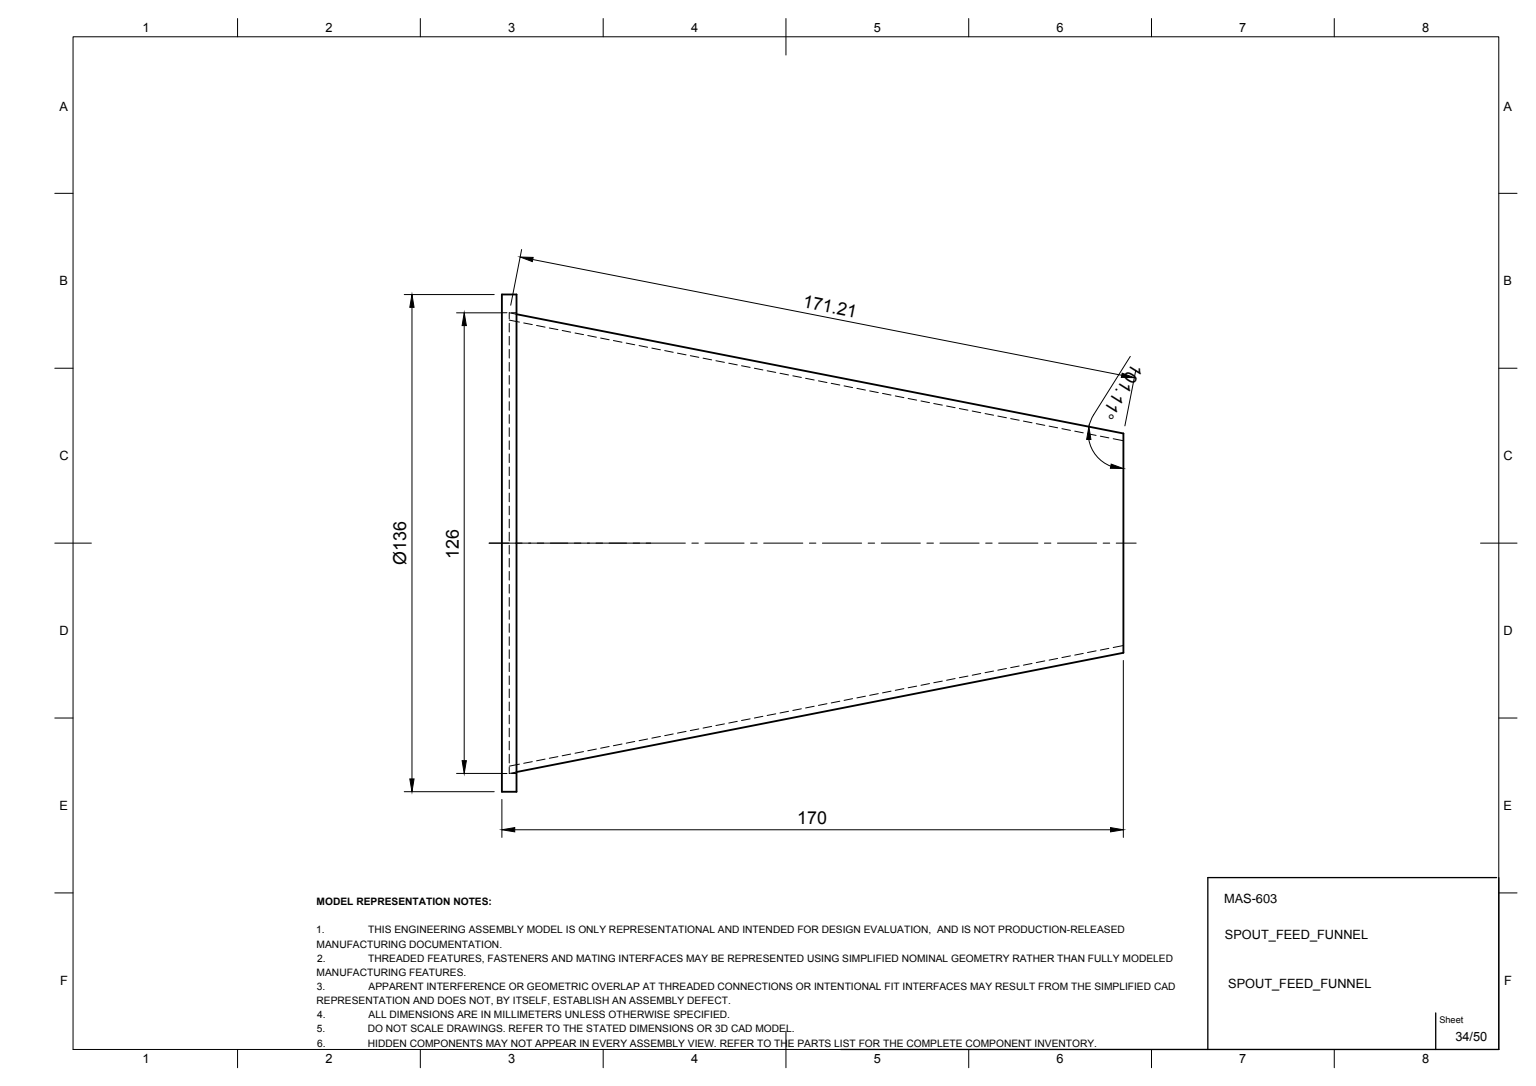
ISO-10303-21;
HEADER;
FILE_DESCRIPTION((''),'2;1');
FILE_NAME('SPOUT_FEED_FUNNEL.step','2026-10-01T22:06:14-07:00',(''),(''),'','','');
FILE_SCHEMA (('AUTOMOTIVE_DESIGN { 1 0 10303 214 3 1 1 }'));
ENDSEC;
DATA;
#10=MECHANICAL_DESIGN_GEOMETRIC_PRESENTATION_REPRESENTATION('',(#1006,#1007),#50440);
#914=SHAPE_REPRESENTATION_RELATIONSHIP('SRR','None',#50647,#959) ;
#959=ADVANCED_BREP_SHAPE_REPRESENTATION('',(#1061,#1062),#50416) ;
#1006=STYLED_ITEM('',(#50889),#1061) ;
#1007=STYLED_ITEM('',(#50889),#1062) ;
#1061=MANIFOLD_SOLID_BREP('SPOUT_FEED_FUNNEL',#28673) ;
#1062=MANIFOLD_SOLID_BREP('SPOUT_FEED_FUNNEL',#28674) ;
#1094=CONICAL_SURFACE('',#30858,4.65,0.193959147259893) ;
#1095=CONICAL_SURFACE('',#30859,4.45,0.193959147259893) ;
#1350=FACE_BOUND('',#5163,.T.) ;
#1351=FACE_BOUND('',#5165,.T.) ;
#1352=FACE_BOUND('',#5167,.T.) ;
#1353=FACE_BOUND('',#5169,.T.) ;
#2201=PLANE('',#30850) ;
#2202=PLANE('',#30851) ;
#2203=PLANE('',#30852) ;
#2204=PLANE('',#30855) ;
#3367=FACE_OUTER_BOUND('',#5159,.T.) ;
#3368=FACE_OUTER_BOUND('',#5160,.T.) ;
#3369=FACE_OUTER_BOUND('',#5161,.T.) ;
#3370=FACE_OUTER_BOUND('',#5162,.T.) ;
#3371=FACE_OUTER_BOUND('',#5164,.T.) ;
#3372=FACE_OUTER_BOUND('',#5166,.T.) ;
#3373=FACE_OUTER_BOUND('',#5168,.T.) ;
#3374=FACE_OUTER_BOUND('',#5170,.T.) ;
#3375=FACE_OUTER_BOUND('',#5171,.T.) ;
#5159=EDGE_LOOP('',(#23895,#23896,#23897,#23898)) ;
#5160=EDGE_LOOP('',(#23899,#23900,#23901,#23902)) ;
#5161=EDGE_LOOP('',(#23903,#23904,#23905,#23906)) ;
#5162=EDGE_LOOP('',(#23907)) ;
#5163=EDGE_LOOP('',(#23908)) ;
#5164=EDGE_LOOP('',(#23909)) ;
#5165=EDGE_LOOP('',(#23910)) ;
#5166=EDGE_LOOP('',(#23911)) ;
#5167=EDGE_LOOP('',(#23912)) ;
#5168=EDGE_LOOP('',(#23913)) ;
#5169=EDGE_LOOP('',(#23914)) ;
#5170=EDGE_LOOP('',(#23915,#23916,#23917,#23918)) ;
#5171=EDGE_LOOP('',(#23919,#23920,#23921,#23922)) ;
#7819=LINE('',#46974,#10291) ;
#7820=LINE('',#46978,#10292) ;
#7821=LINE('',#46984,#10293) ;
#7822=LINE('',#46999,#10294) ;
#7823=LINE('',#47001,#10295) ;
#10291=VECTOR('',#37732,6.3) ;
#10292=VECTOR('',#37737,6.3) ;
#10293=VECTOR('',#37744,6.8) ;
#10294=VECTOR('',#37765,4.65) ;
#10295=VECTOR('',#37768,4.45) ;
#11196=CIRCLE('',#30843,6.3) ;
#11197=CIRCLE('',#30844,6.3) ;
#11198=CIRCLE('',#30846,6.3) ;
#11199=CIRCLE('',#30848,6.8) ;
#11200=CIRCLE('',#30849,6.8) ;
#11201=CIRCLE('',#30853,3.) ;
#11202=CIRCLE('',#30854,2.8) ;
#11203=CIRCLE('',#30856,6.3) ;
#11204=CIRCLE('',#30857,6.1) ;
#13614=VERTEX_POINT('',#46971) ;
#13615=VERTEX_POINT('',#46973) ;
#13616=VERTEX_POINT('',#46977) ;
#13617=VERTEX_POINT('',#46981) ;
#13618=VERTEX_POINT('',#46983) ;
#13619=VERTEX_POINT('',#46989) ;
#13620=VERTEX_POINT('',#46991) ;
#13621=VERTEX_POINT('',#46994) ;
#13622=VERTEX_POINT('',#46996) ;
#17213=EDGE_CURVE('',#13614,#13614,#11196,.T.) ;
#17214=EDGE_CURVE('',#13614,#13615,#7819,.T.) ;
#17215=EDGE_CURVE('',#13615,#13615,#11197,.T.) ;
#17216=EDGE_CURVE('',#13615,#13616,#7820,.T.) ;
#17217=EDGE_CURVE('',#13616,#13616,#11198,.T.) ;
#17218=EDGE_CURVE('',#13617,#13617,#11199,.T.) ;
#17219=EDGE_CURVE('',#13617,#13618,#7821,.T.) ;
#17220=EDGE_CURVE('',#13618,#13618,#11200,.T.) ;
#17221=EDGE_CURVE('',#13619,#13619,#11201,.T.) ;
#17222=EDGE_CURVE('',#13620,#13620,#11202,.T.) ;
#17223=EDGE_CURVE('',#13621,#13621,#11203,.T.) ;
#17224=EDGE_CURVE('',#13622,#13622,#11204,.T.) ;
#17225=EDGE_CURVE('',#13619,#13621,#7822,.T.) ;
#17226=EDGE_CURVE('',#13622,#13620,#7823,.T.) ;
#23895=ORIENTED_EDGE('',*,*,#17213,.F.) ;
#23896=ORIENTED_EDGE('',*,*,#17214,.T.) ;
#23897=ORIENTED_EDGE('',*,*,#17215,.T.) ;
#23898=ORIENTED_EDGE('',*,*,#17214,.F.) ;
#23899=ORIENTED_EDGE('',*,*,#17215,.F.) ;
#23900=ORIENTED_EDGE('',*,*,#17216,.T.) ;
#23901=ORIENTED_EDGE('',*,*,#17217,.F.) ;
#23902=ORIENTED_EDGE('',*,*,#17216,.F.) ;
#23903=ORIENTED_EDGE('',*,*,#17218,.F.) ;
#23904=ORIENTED_EDGE('',*,*,#17219,.T.) ;
#23905=ORIENTED_EDGE('',*,*,#17220,.F.) ;
#23906=ORIENTED_EDGE('',*,*,#17219,.F.) ;
#23907=ORIENTED_EDGE('',*,*,#17220,.T.) ;
#23908=ORIENTED_EDGE('',*,*,#17213,.T.) ;
#23909=ORIENTED_EDGE('',*,*,#17218,.T.) ;
#23910=ORIENTED_EDGE('',*,*,#17217,.T.) ;
#23911=ORIENTED_EDGE('',*,*,#17221,.T.) ;
#23912=ORIENTED_EDGE('',*,*,#17222,.T.) ;
#23913=ORIENTED_EDGE('',*,*,#17223,.T.) ;
#23914=ORIENTED_EDGE('',*,*,#17224,.T.) ;
#23915=ORIENTED_EDGE('',*,*,#17221,.F.) ;
#23916=ORIENTED_EDGE('',*,*,#17225,.T.) ;
#23917=ORIENTED_EDGE('',*,*,#17223,.F.) ;
#23918=ORIENTED_EDGE('',*,*,#17225,.F.) ;
#23919=ORIENTED_EDGE('',*,*,#17224,.F.) ;
#23920=ORIENTED_EDGE('',*,*,#17226,.T.) ;
#23921=ORIENTED_EDGE('',*,*,#17222,.F.) ;
#23922=ORIENTED_EDGE('',*,*,#17226,.F.) ;
#26853=CYLINDRICAL_SURFACE('',#30842,6.3) ;
#26854=CYLINDRICAL_SURFACE('',#30845,6.3) ;
#26855=CYLINDRICAL_SURFACE('',#30847,6.8) ;
#28102=ADVANCED_FACE('',(#3367),#26853,.F.) ;
#28103=ADVANCED_FACE('',(#3368),#26854,.F.) ;
#28104=ADVANCED_FACE('',(#3369),#26855,.T.) ;
#28105=ADVANCED_FACE('',(#3370,#1350),#2201,.T.) ;
#28106=ADVANCED_FACE('',(#3371,#1351),#2202,.T.) ;
#28107=ADVANCED_FACE('',(#3372,#1352),#2203,.T.) ;
#28108=ADVANCED_FACE('',(#3373,#1353),#2204,.T.) ;
#28109=ADVANCED_FACE('',(#3374),#1094,.T.) ;
#28110=ADVANCED_FACE('',(#3375),#1095,.F.) ;
#28673=CLOSED_SHELL('',(#28102,#28103,#28104,#28105,#28106)) ;
#28674=CLOSED_SHELL('',(#28107,#28108,#28109,#28110)) ;
#30841=AXIS2_PLACEMENT_3D('',#46969,#37726,#37727) ;
#30842=AXIS2_PLACEMENT_3D('',#46970,#37728,#37729) ;
#30843=AXIS2_PLACEMENT_3D('',#46972,#37730,#37731) ;
#30844=AXIS2_PLACEMENT_3D('',#46975,#37733,#37734) ;
#30845=AXIS2_PLACEMENT_3D('',#46976,#37735,#37736) ;
#30846=AXIS2_PLACEMENT_3D('',#46979,#37738,#37739) ;
#30847=AXIS2_PLACEMENT_3D('',#46980,#37740,#37741) ;
#30848=AXIS2_PLACEMENT_3D('',#46982,#37742,#37743) ;
#30849=AXIS2_PLACEMENT_3D('',#46985,#37745,#37746) ;
#30850=AXIS2_PLACEMENT_3D('',#46986,#37747,#37748) ;
#30851=AXIS2_PLACEMENT_3D('',#46987,#37749,#37750) ;
#30852=AXIS2_PLACEMENT_3D('',#46988,#37751,#37752) ;
#30853=AXIS2_PLACEMENT_3D('',#46990,#37753,#37754) ;
#30854=AXIS2_PLACEMENT_3D('',#46992,#37755,#37756) ;
#30855=AXIS2_PLACEMENT_3D('',#46993,#37757,#37758) ;
#30856=AXIS2_PLACEMENT_3D('',#46995,#37759,#37760) ;
#30857=AXIS2_PLACEMENT_3D('',#46997,#37761,#37762) ;
#30858=AXIS2_PLACEMENT_3D('',#46998,#37763,#37764) ;
#30859=AXIS2_PLACEMENT_3D('',#47000,#37766,#37767) ;
#37726=DIRECTION('axis',(0.,0.,1.)) ;
#37727=DIRECTION('refdir',(1.,0.,0.)) ;
#37728=DIRECTION('center_axis',(0.,0.,1.)) ;
#37729=DIRECTION('ref_axis',(1.,0.,0.)) ;
#37730=DIRECTION('center_axis',(0.,0.,1.)) ;
#37731=DIRECTION('ref_axis',(1.,0.,0.)) ;
#37732=DIRECTION('',(0.,0.,1.)) ;
#37733=DIRECTION('center_axis',(0.,0.,1.)) ;
#37734=DIRECTION('ref_axis',(1.,0.,0.)) ;
#37735=DIRECTION('center_axis',(0.,0.,1.)) ;
#37736=DIRECTION('ref_axis',(1.,0.,0.)) ;
#37737=DIRECTION('',(0.,0.,1.)) ;
#37738=DIRECTION('center_axis',(0.,0.,-1.)) ;
#37739=DIRECTION('ref_axis',(1.,0.,0.)) ;
#37740=DIRECTION('center_axis',(0.,0.,1.)) ;
#37741=DIRECTION('ref_axis',(1.,0.,0.)) ;
#37742=DIRECTION('center_axis',(0.,0.,1.)) ;
#37743=DIRECTION('ref_axis',(1.,0.,0.)) ;
#37744=DIRECTION('',(0.,0.,-1.)) ;
#37745=DIRECTION('center_axis',(0.,0.,-1.)) ;
#37746=DIRECTION('ref_axis',(1.,0.,0.)) ;
#37747=DIRECTION('center_axis',(0.,0.,-1.)) ;
#37748=DIRECTION('ref_axis',(-1.,0.,0.)) ;
#37749=DIRECTION('center_axis',(0.,0.,1.)) ;
#37750=DIRECTION('ref_axis',(1.,0.,0.)) ;
#37751=DIRECTION('center_axis',(0.,0.,-1.)) ;
#37752=DIRECTION('ref_axis',(1.,0.,0.)) ;
#37753=DIRECTION('center_axis',(0.,0.,-1.)) ;
#37754=DIRECTION('ref_axis',(1.,0.,0.)) ;
#37755=DIRECTION('center_axis',(0.,0.,1.)) ;
#37756=DIRECTION('ref_axis',(1.,0.,0.)) ;
#37757=DIRECTION('center_axis',(0.,0.,1.)) ;
#37758=DIRECTION('ref_axis',(-1.,0.,0.)) ;
#37759=DIRECTION('center_axis',(0.,0.,1.)) ;
#37760=DIRECTION('ref_axis',(1.,0.,0.)) ;
#37761=DIRECTION('center_axis',(0.,0.,-1.)) ;
#37762=DIRECTION('ref_axis',(1.,0.,0.)) ;
#37763=DIRECTION('center_axis',(0.,0.,1.)) ;
#37764=DIRECTION('ref_axis',(1.,0.,0.)) ;
#37765=DIRECTION('',(-0.192745304030928,2.36044919632159E-17,0.981248820521087)) ;
#37766=DIRECTION('center_axis',(0.,0.,1.)) ;
#37767=DIRECTION('ref_axis',(1.,0.,0.)) ;
#37768=DIRECTION('',(0.192745304030928,-2.36044919632159E-17,-0.981248820521087)) ;
#46969=CARTESIAN_POINT('',(0.,0.,0.)) ;
#46970=CARTESIAN_POINT('Origin',(0.,0.,41.8)) ;
#46971=CARTESIAN_POINT('',(-6.3,-7.71527483462833E-16,41.6)) ;
#46972=CARTESIAN_POINT('Origin',(0.,0.,41.6)) ;
#46973=CARTESIAN_POINT('',(-6.3,-7.71527483462833E-16,41.8)) ;
#46974=CARTESIAN_POINT('',(-6.3,-7.71527483462833E-16,41.8)) ;
#46975=CARTESIAN_POINT('Origin',(0.,0.,41.8)) ;
#46976=CARTESIAN_POINT('Origin',(0.,0.,41.8)) ;
#46977=CARTESIAN_POINT('',(-6.3,7.71527483462833E-16,42.)) ;
#46978=CARTESIAN_POINT('',(-6.3,-7.71527483462833E-16,41.8)) ;
#46979=CARTESIAN_POINT('Origin',(0.,0.,42.)) ;
#46980=CARTESIAN_POINT('Origin',(0.,0.,41.8)) ;
#46981=CARTESIAN_POINT('',(-6.8,-8.327598234202E-16,42.)) ;
#46982=CARTESIAN_POINT('Origin',(0.,0.,42.)) ;
#46983=CARTESIAN_POINT('',(-6.8,-8.327598234202E-16,41.6)) ;
#46984=CARTESIAN_POINT('',(-6.8,-8.327598234202E-16,41.8)) ;
#46985=CARTESIAN_POINT('Origin',(0.,0.,41.6)) ;
#46986=CARTESIAN_POINT('Origin',(0.,0.,41.6)) ;
#46987=CARTESIAN_POINT('Origin',(0.,0.,42.)) ;
#46988=CARTESIAN_POINT('Origin',(0.,0.,25.)) ;
#46989=CARTESIAN_POINT('',(-3.,3.67394039744206E-16,25.)) ;
#46990=CARTESIAN_POINT('Origin',(0.,0.,25.)) ;
#46991=CARTESIAN_POINT('',(-2.8,-3.42901103761259E-16,25.)) ;
#46992=CARTESIAN_POINT('Origin',(0.,0.,25.)) ;
#46993=CARTESIAN_POINT('Origin',(0.,0.,41.8)) ;
#46994=CARTESIAN_POINT('',(-6.3,-7.71527483462833E-16,41.8)) ;
#46995=CARTESIAN_POINT('Origin',(0.,0.,41.8)) ;
#46996=CARTESIAN_POINT('',(-6.1,7.47034547479886E-16,41.8)) ;
#46997=CARTESIAN_POINT('Origin',(0.,0.,41.8)) ;
#46998=CARTESIAN_POINT('Origin',(0.,0.,33.4)) ;
#46999=CARTESIAN_POINT('',(-4.65,5.69460761603519E-16,33.4)) ;
#47000=CARTESIAN_POINT('Origin',(0.,0.,33.4)) ;
#47001=CARTESIAN_POINT('',(-4.45,5.44967825620572E-16,33.4)) ;
#50363=UNCERTAINTY_MEASURE_WITH_UNIT(LENGTH_MEASURE(0.001),#50441,
'DISTANCE_ACCURACY_VALUE',
'Maximum model space distance between geometric entities at asserted c
onnectivities') ;
#50387=UNCERTAINTY_MEASURE_WITH_UNIT(LENGTH_MEASURE(0.001),#50441,
'DISTANCE_ACCURACY_VALUE',
'Maximum model space distance between geometric entities at asserted c
onnectivities') ;
#50416=(
GEOMETRIC_REPRESENTATION_CONTEXT(3)
GLOBAL_UNCERTAINTY_ASSIGNED_CONTEXT((#50363))
GLOBAL_UNIT_ASSIGNED_CONTEXT((#50441,#50443,#50444))
REPRESENTATION_CONTEXT('','3D')
) ;
#50440=(
GEOMETRIC_REPRESENTATION_CONTEXT(3)
GLOBAL_UNCERTAINTY_ASSIGNED_CONTEXT((#50387))
GLOBAL_UNIT_ASSIGNED_CONTEXT((#50441,#50443,#50444))
REPRESENTATION_CONTEXT('','3D')
) ;
#50441=(
LENGTH_UNIT()
NAMED_UNIT(*)
SI_UNIT(.CENTI.,.METRE.)
) ;
#50443=(
NAMED_UNIT(*)
PLANE_ANGLE_UNIT()
SI_UNIT($,.RADIAN.)
) ;
#50444=(
NAMED_UNIT(*)
SI_UNIT($,.STERADIAN.)
SOLID_ANGLE_UNIT()
) ;
#50473=SHAPE_DEFINITION_REPRESENTATION(#50549,#50647) ;
#50549=PRODUCT_DEFINITION_SHAPE('',$,#50700) ;
#50647=SHAPE_REPRESENTATION('',(#30841),#50416) ;
#50671=PRODUCT_DEFINITION_CONTEXT('part definition',#50829,'design') ;
#50700=PRODUCT_DEFINITION('SPOUT_FEED_FUNNEL','SPOUT_FEED_FUNNEL',
#50752,#50671) ;
#50752=PRODUCT_DEFINITION_FORMATION('',$,#50859) ;
#50829=APPLICATION_CONTEXT(
'Core Data for Automotive Mechanical Design Process') ;
#50830=PRODUCT_CONTEXT('part definition',#50829,'mechanical') ;
#50859=PRODUCT('SPOUT_FEED_FUNNEL','SPOUT_FEED_FUNNEL',$,(#50830)) ;
#50889=PRESENTATION_STYLE_ASSIGNMENT((#50896)) ;
#50896=SURFACE_STYLE_USAGE(.BOTH.,#50903) ;
#50903=SURFACE_SIDE_STYLE('',(#50910)) ;
#50910=SURFACE_STYLE_FILL_AREA(#50917) ;
#50917=FILL_AREA_STYLE('Stainless Steel - Satin',(#50924)) ;
#50924=FILL_AREA_STYLE_COLOUR('Stainless Steel - Satin',#50931) ;
#50931=COLOUR_RGB('Stainless Steel - Satin', 0.72549020, 0.75294118, 0.79215686) ;
ENDSEC;
END-ISO-10303-21;
